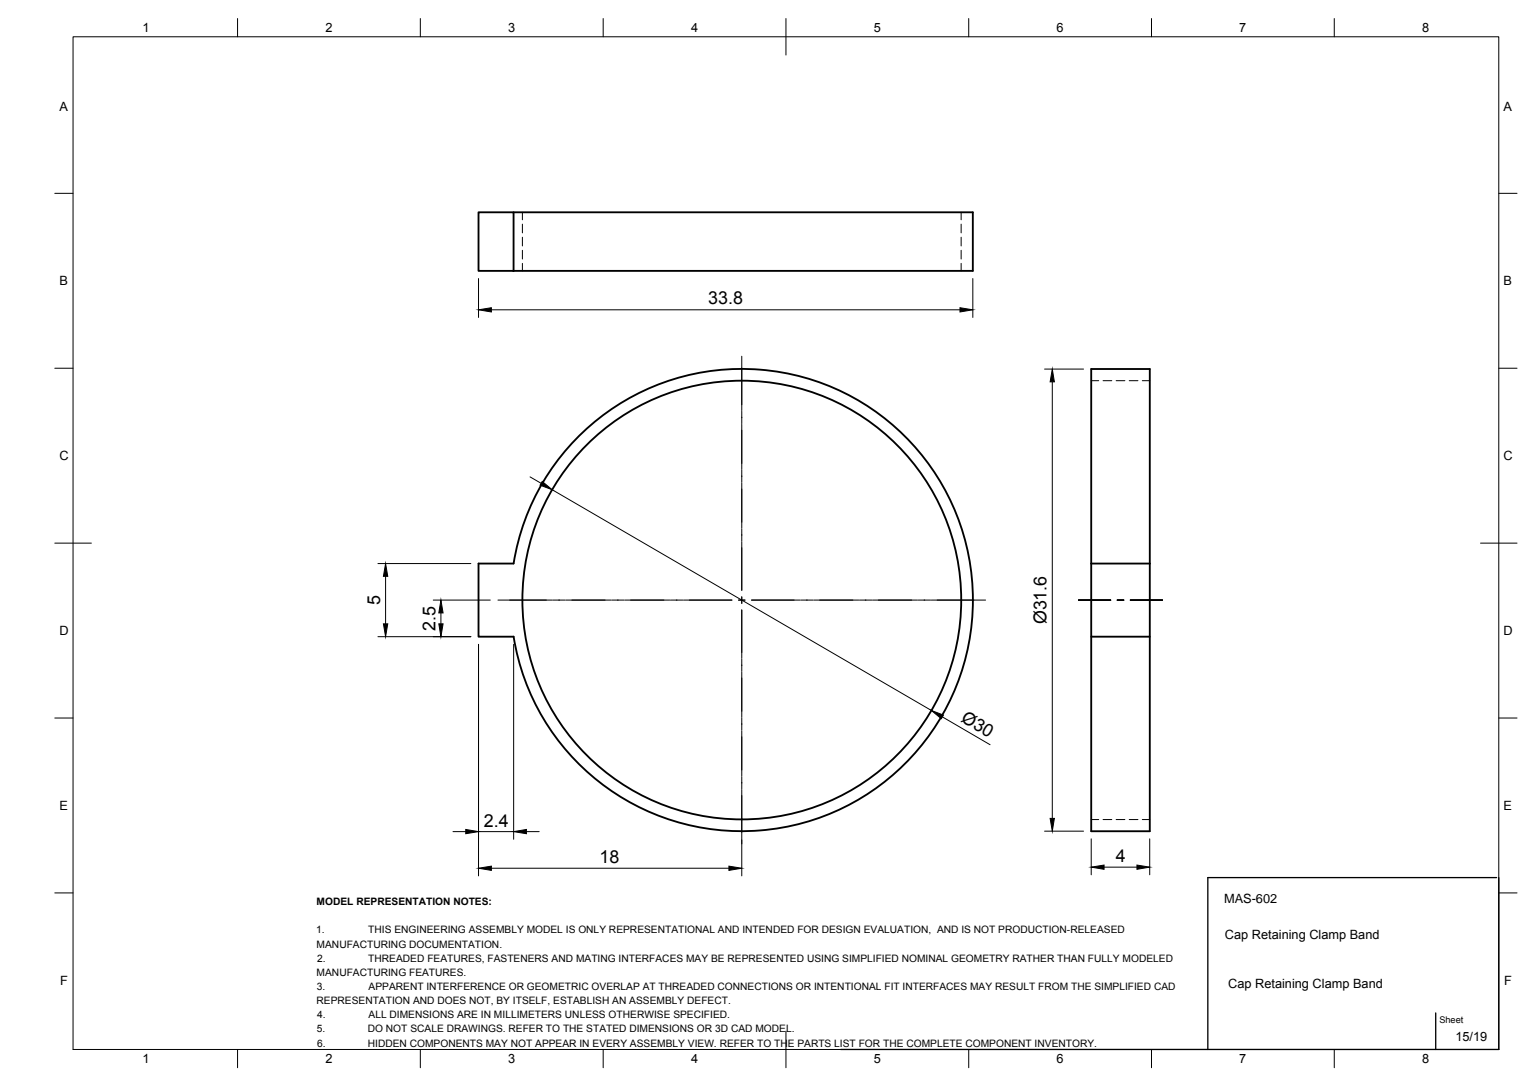
ISO-10303-21;
HEADER;
/* Generated by software containing ST-Developer
 * from STEP Tools, Inc. (www.steptools.com) 
 */

FILE_DESCRIPTION(
/* description */ (''),
/* implementation_level */ '2;1');

FILE_NAME(
/* name */ 'Cap Retaining Clamp Band.step',
/* time_stamp */ '2026-10-15T14:42:47-07:00',
/* author */ (''),
/* organization */ (''),
/* preprocessor_version */ 'ST-DEVELOPER v20.2',
/* originating_system */ 'Autodesk Translation Framework v15.15.0.0',
/* authorisation */ '');

FILE_SCHEMA (('AUTOMOTIVE_DESIGN { 1 0 10303 214 3 1 1 }'));
ENDSEC;

DATA;
#10=MECHANICAL_DESIGN_GEOMETRIC_PRESENTATION_REPRESENTATION('',(#243),#85789);
#207=SHAPE_REPRESENTATION_RELATIONSHIP('SRR','None',#85872,#225);
#225=ADVANCED_BREP_SHAPE_REPRESENTATION('',(#261),#85780);
#243=STYLED_ITEM('',(#85971),#261);
#261=MANIFOLD_SOLID_BREP('Body1',#9890);
#459=FACE_BOUND('',#3357,.T.);
#460=FACE_BOUND('',#3361,.T.);
#1154=PLANE('',#10680);
#1155=PLANE('',#10681);
#1156=PLANE('',#10682);
#1157=PLANE('',#10683);
#1158=PLANE('',#10690);
#1623=LINE('',#77692,#2159);
#1624=LINE('',#77694,#2160);
#1625=LINE('',#77696,#2161);
#1626=LINE('',#77697,#2162);
#1627=LINE('',#77701,#2163);
#1628=LINE('',#77703,#2164);
#1629=LINE('',#77705,#2165);
#1630=LINE('',#77706,#2166);
#1631=LINE('',#77708,#2167);
#1632=LINE('',#77709,#2168);
#1633=LINE('',#77717,#2169);
#2159=VECTOR('',#12549,1.);
#2160=VECTOR('',#12550,1.);
#2161=VECTOR('',#12551,1.);
#2162=VECTOR('',#12552,1.);
#2163=VECTOR('',#12555,1.);
#2164=VECTOR('',#12556,1.);
#2165=VECTOR('',#12557,1.);
#2166=VECTOR('',#12558,1.);
#2167=VECTOR('',#12561,1.);
#2168=VECTOR('',#12562,1.);
#2169=VECTOR('',#12573,1.5);
#2348=CYLINDRICAL_SURFACE('',#10686,1.5);
#2349=CYLINDRICAL_SURFACE('',#10688,1.58);
#2779=FACE_OUTER_BOUND('',#3353,.T.);
#2780=FACE_OUTER_BOUND('',#3354,.T.);
#2781=FACE_OUTER_BOUND('',#3355,.T.);
#2782=FACE_OUTER_BOUND('',#3356,.T.);
#2783=FACE_OUTER_BOUND('',#3358,.T.);
#2784=FACE_OUTER_BOUND('',#3359,.T.);
#2785=FACE_OUTER_BOUND('',#3360,.T.);
#3353=EDGE_LOOP('',(#8727,#8728,#8729,#8730));
#3354=EDGE_LOOP('',(#8731,#8732,#8733,#8734));
#3355=EDGE_LOOP('',(#8735,#8736,#8737,#8738));
#3356=EDGE_LOOP('',(#8739,#8740,#8741,#8742));
#3357=EDGE_LOOP('',(#8743));
#3358=EDGE_LOOP('',(#8744,#8745,#8746,#8747));
#3359=EDGE_LOOP('',(#8748,#8749,#8750,#8751));
#3360=EDGE_LOOP('',(#8752,#8753,#8754,#8755));
#3361=EDGE_LOOP('',(#8756));
#3776=CIRCLE('',#10684,1.58);
#3777=CIRCLE('',#10685,1.5);
#3778=CIRCLE('',#10687,1.5);
#3779=CIRCLE('',#10689,1.58);
#4707=VERTEX_POINT('',#77690);
#4708=VERTEX_POINT('',#77691);
#4709=VERTEX_POINT('',#77693);
#4710=VERTEX_POINT('',#77695);
#4711=VERTEX_POINT('',#77699);
#4712=VERTEX_POINT('',#77700);
#4713=VERTEX_POINT('',#77702);
#4714=VERTEX_POINT('',#77704);
#4715=VERTEX_POINT('',#77712);
#4716=VERTEX_POINT('',#77715);
#6091=EDGE_CURVE('',#4707,#4708,#1623,.T.);
#6092=EDGE_CURVE('',#4707,#4709,#1624,.T.);
#6093=EDGE_CURVE('',#4709,#4710,#1625,.T.);
#6094=EDGE_CURVE('',#4708,#4710,#1626,.T.);
#6095=EDGE_CURVE('',#4711,#4712,#1627,.T.);
#6096=EDGE_CURVE('',#4713,#4711,#1628,.T.);
#6097=EDGE_CURVE('',#4714,#4713,#1629,.T.);
#6098=EDGE_CURVE('',#4714,#4712,#1630,.T.);
#6099=EDGE_CURVE('',#4709,#4714,#1631,.T.);
#6100=EDGE_CURVE('',#4710,#4713,#1632,.T.);
#6101=EDGE_CURVE('',#4711,#4708,#3776,.T.);
#6102=EDGE_CURVE('',#4715,#4715,#3777,.T.);
#6103=EDGE_CURVE('',#4716,#4716,#3778,.T.);
#6104=EDGE_CURVE('',#4716,#4715,#1633,.T.);
#6105=EDGE_CURVE('',#4712,#4707,#3779,.T.);
#8727=ORIENTED_EDGE('',*,*,#6091,.F.);
#8728=ORIENTED_EDGE('',*,*,#6092,.T.);
#8729=ORIENTED_EDGE('',*,*,#6093,.T.);
#8730=ORIENTED_EDGE('',*,*,#6094,.F.);
#8731=ORIENTED_EDGE('',*,*,#6095,.F.);
#8732=ORIENTED_EDGE('',*,*,#6096,.F.);
#8733=ORIENTED_EDGE('',*,*,#6097,.F.);
#8734=ORIENTED_EDGE('',*,*,#6098,.T.);
#8735=ORIENTED_EDGE('',*,*,#6099,.T.);
#8736=ORIENTED_EDGE('',*,*,#6097,.T.);
#8737=ORIENTED_EDGE('',*,*,#6100,.F.);
#8738=ORIENTED_EDGE('',*,*,#6093,.F.);
#8739=ORIENTED_EDGE('',*,*,#6101,.T.);
#8740=ORIENTED_EDGE('',*,*,#6094,.T.);
#8741=ORIENTED_EDGE('',*,*,#6100,.T.);
#8742=ORIENTED_EDGE('',*,*,#6096,.T.);
#8743=ORIENTED_EDGE('',*,*,#6102,.T.);
#8744=ORIENTED_EDGE('',*,*,#6103,.T.);
#8745=ORIENTED_EDGE('',*,*,#6104,.T.);
#8746=ORIENTED_EDGE('',*,*,#6102,.F.);
#8747=ORIENTED_EDGE('',*,*,#6104,.F.);
#8748=ORIENTED_EDGE('',*,*,#6091,.T.);
#8749=ORIENTED_EDGE('',*,*,#6101,.F.);
#8750=ORIENTED_EDGE('',*,*,#6095,.T.);
#8751=ORIENTED_EDGE('',*,*,#6105,.T.);
#8752=ORIENTED_EDGE('',*,*,#6105,.F.);
#8753=ORIENTED_EDGE('',*,*,#6098,.F.);
#8754=ORIENTED_EDGE('',*,*,#6099,.F.);
#8755=ORIENTED_EDGE('',*,*,#6092,.F.);
#8756=ORIENTED_EDGE('',*,*,#6103,.F.);
#9757=ADVANCED_FACE('',(#2779),#1154,.T.);
#9758=ADVANCED_FACE('',(#2780),#1155,.T.);
#9759=ADVANCED_FACE('',(#2781),#1156,.T.);
#9760=ADVANCED_FACE('',(#2782,#459),#1157,.T.);
#9761=ADVANCED_FACE('',(#2783),#2348,.F.);
#9762=ADVANCED_FACE('',(#2784),#2349,.T.);
#9763=ADVANCED_FACE('',(#2785,#460),#1158,.F.);
#9890=CLOSED_SHELL('',(#9757,#9758,#9759,#9760,#9761,#9762,#9763));
#10679=AXIS2_PLACEMENT_3D('',#77688,#12545,#12546);
#10680=AXIS2_PLACEMENT_3D('',#77689,#12547,#12548);
#10681=AXIS2_PLACEMENT_3D('',#77698,#12553,#12554);
#10682=AXIS2_PLACEMENT_3D('',#77707,#12559,#12560);
#10683=AXIS2_PLACEMENT_3D('',#77710,#12563,#12564);
#10684=AXIS2_PLACEMENT_3D('',#77711,#12565,#12566);
#10685=AXIS2_PLACEMENT_3D('',#77713,#12567,#12568);
#10686=AXIS2_PLACEMENT_3D('',#77714,#12569,#12570);
#10687=AXIS2_PLACEMENT_3D('',#77716,#12571,#12572);
#10688=AXIS2_PLACEMENT_3D('',#77718,#12574,#12575);
#10689=AXIS2_PLACEMENT_3D('',#77719,#12576,#12577);
#10690=AXIS2_PLACEMENT_3D('',#77720,#12578,#12579);
#12545=DIRECTION('axis',(0.,0.,1.));
#12546=DIRECTION('refdir',(1.,0.,0.));
#12547=DIRECTION('center_axis',(1.,0.,0.));
#12548=DIRECTION('ref_axis',(0.,1.,0.));
#12549=DIRECTION('',(0.,0.,1.));
#12550=DIRECTION('',(0.,1.,0.));
#12551=DIRECTION('',(0.,0.,1.));
#12552=DIRECTION('',(0.,1.,0.));
#12553=DIRECTION('center_axis',(-1.,0.,0.));
#12554=DIRECTION('ref_axis',(0.,-1.,0.));
#12555=DIRECTION('',(0.,0.,-1.));
#12556=DIRECTION('',(0.,-1.,0.));
#12557=DIRECTION('',(0.,0.,1.));
#12558=DIRECTION('',(0.,-1.,0.));
#12559=DIRECTION('center_axis',(0.,1.,0.));
#12560=DIRECTION('ref_axis',(-1.,0.,0.));
#12561=DIRECTION('',(-1.,0.,0.));
#12562=DIRECTION('',(-1.,0.,0.));
#12563=DIRECTION('center_axis',(0.,0.,1.));
#12564=DIRECTION('ref_axis',(1.,0.,0.));
#12565=DIRECTION('center_axis',(0.,0.,1.));
#12566=DIRECTION('ref_axis',(1.,0.,0.));
#12567=DIRECTION('center_axis',(0.,0.,-1.));
#12568=DIRECTION('ref_axis',(1.,0.,0.));
#12569=DIRECTION('center_axis',(0.,0.,1.));
#12570=DIRECTION('ref_axis',(1.,0.,0.));
#12571=DIRECTION('center_axis',(0.,0.,-1.));
#12572=DIRECTION('ref_axis',(1.,0.,0.));
#12573=DIRECTION('',(0.,0.,1.));
#12574=DIRECTION('center_axis',(0.,0.,1.));
#12575=DIRECTION('ref_axis',(6.12323399573677E-17,-1.,0.));
#12576=DIRECTION('center_axis',(0.,0.,1.));
#12577=DIRECTION('ref_axis',(1.,0.,0.));
#12578=DIRECTION('center_axis',(0.,0.,1.));
#12579=DIRECTION('ref_axis',(1.,0.,0.));
#77688=CARTESIAN_POINT('',(0.,0.,0.));
#77689=CARTESIAN_POINT('Origin',(0.25,3.66,12.85));
#77690=CARTESIAN_POINT('',(0.25,3.66009615088302,12.85));
#77691=CARTESIAN_POINT('',(0.25,3.66009615088302,13.25));
#77692=CARTESIAN_POINT('',(0.25,3.66009615088302,12.85));
#77693=CARTESIAN_POINT('',(0.25,3.9,12.85));
#77694=CARTESIAN_POINT('',(0.25,3.66,12.85));
#77695=CARTESIAN_POINT('',(0.25,3.9,13.25));
#77696=CARTESIAN_POINT('',(0.25,3.9,12.85));
#77697=CARTESIAN_POINT('',(0.25,3.66,13.25));
#77698=CARTESIAN_POINT('Origin',(-0.25,3.9,12.85));
#77699=CARTESIAN_POINT('',(-0.25,3.66009615088302,13.25));
#77700=CARTESIAN_POINT('',(-0.25,3.66009615088302,12.85));
#77701=CARTESIAN_POINT('',(-0.25,3.66009615088302,12.85));
#77702=CARTESIAN_POINT('',(-0.25,3.9,13.25));
#77703=CARTESIAN_POINT('',(-0.25,3.9,13.25));
#77704=CARTESIAN_POINT('',(-0.25,3.9,12.85));
#77705=CARTESIAN_POINT('',(-0.25,3.9,12.85));
#77706=CARTESIAN_POINT('',(-0.25,3.9,12.85));
#77707=CARTESIAN_POINT('Origin',(0.25,3.9,12.85));
#77708=CARTESIAN_POINT('',(0.25,3.9,12.85));
#77709=CARTESIAN_POINT('',(0.25,3.9,13.25));
#77710=CARTESIAN_POINT('Origin',(0.,2.1,13.25));
#77711=CARTESIAN_POINT('Origin',(0.,2.1,13.25));
#77712=CARTESIAN_POINT('',(-1.5,2.1,13.25));
#77713=CARTESIAN_POINT('Origin',(0.,2.1,13.25));
#77714=CARTESIAN_POINT('Origin',(0.,2.1,12.85));
#77715=CARTESIAN_POINT('',(-1.5,2.1,12.85));
#77716=CARTESIAN_POINT('Origin',(0.,2.1,12.85));
#77717=CARTESIAN_POINT('',(-1.5,2.1,12.85));
#77718=CARTESIAN_POINT('Origin',(0.,2.1,12.85));
#77719=CARTESIAN_POINT('Origin',(0.,2.1,12.85));
#77720=CARTESIAN_POINT('Origin',(0.,2.1,12.85));
#85760=UNCERTAINTY_MEASURE_WITH_UNIT(LENGTH_MEASURE(0.001),#85790,
'DISTANCE_ACCURACY_VALUE',
'Maximum model space distance between geometric entities at asserted c
onnectivities');
#85769=UNCERTAINTY_MEASURE_WITH_UNIT(LENGTH_MEASURE(0.001),#85790,
'DISTANCE_ACCURACY_VALUE',
'Maximum model space distance between geometric entities at asserted c
onnectivities');
#85780=(
GEOMETRIC_REPRESENTATION_CONTEXT(3)
GLOBAL_UNCERTAINTY_ASSIGNED_CONTEXT((#85760))
GLOBAL_UNIT_ASSIGNED_CONTEXT((#85790,#85792,#85793))
REPRESENTATION_CONTEXT('','3D')
);
#85789=(
GEOMETRIC_REPRESENTATION_CONTEXT(3)
GLOBAL_UNCERTAINTY_ASSIGNED_CONTEXT((#85769))
GLOBAL_UNIT_ASSIGNED_CONTEXT((#85790,#85792,#85793))
REPRESENTATION_CONTEXT('','3D')
);
#85790=(
LENGTH_UNIT()
NAMED_UNIT(*)
SI_UNIT(.CENTI.,.METRE.)
);
#85792=(
NAMED_UNIT(*)
PLANE_ANGLE_UNIT()
SI_UNIT($,.RADIAN.)
);
#85793=(
NAMED_UNIT(*)
SI_UNIT($,.STERADIAN.)
SOLID_ANGLE_UNIT()
);
#85804=SHAPE_DEFINITION_REPRESENTATION(#85823,#85872);
#85823=PRODUCT_DEFINITION_SHAPE('',$,#85892);
#85872=SHAPE_REPRESENTATION('',(#10679),#85780);
#85881=PRODUCT_DEFINITION_CONTEXT('part definition',#85940,'design');
#85892=PRODUCT_DEFINITION('Cap Retaining Clamp Band',
'Cap Retaining Clamp Band',#85911,#85881);
#85911=PRODUCT_DEFINITION_FORMATION('',$,#85952);
#85940=APPLICATION_CONTEXT(
'Core Data for Automotive Mechanical Design Process');
#85941=PRODUCT_CONTEXT('part definition',#85940,'mechanical');
#85952=PRODUCT('Cap Retaining Clamp Band','Cap Retaining Clamp Band',$,
(#85941));
#85971=PRESENTATION_STYLE_ASSIGNMENT((#85989));
#85989=SURFACE_STYLE_USAGE(.BOTH.,#86007);
#86007=SURFACE_SIDE_STYLE('',(#86025));
#86025=SURFACE_STYLE_FILL_AREA(#86043);
#86043=FILL_AREA_STYLE('Opaque(205,208,212)',(#86061));
#86061=FILL_AREA_STYLE_COLOUR('Opaque(205,208,212)',#86079);
#86079=COLOUR_RGB('Opaque(205,208,212)', 0.72549020, 0.75294118, 0.79215686);
ENDSEC;
END-ISO-10303-21;
